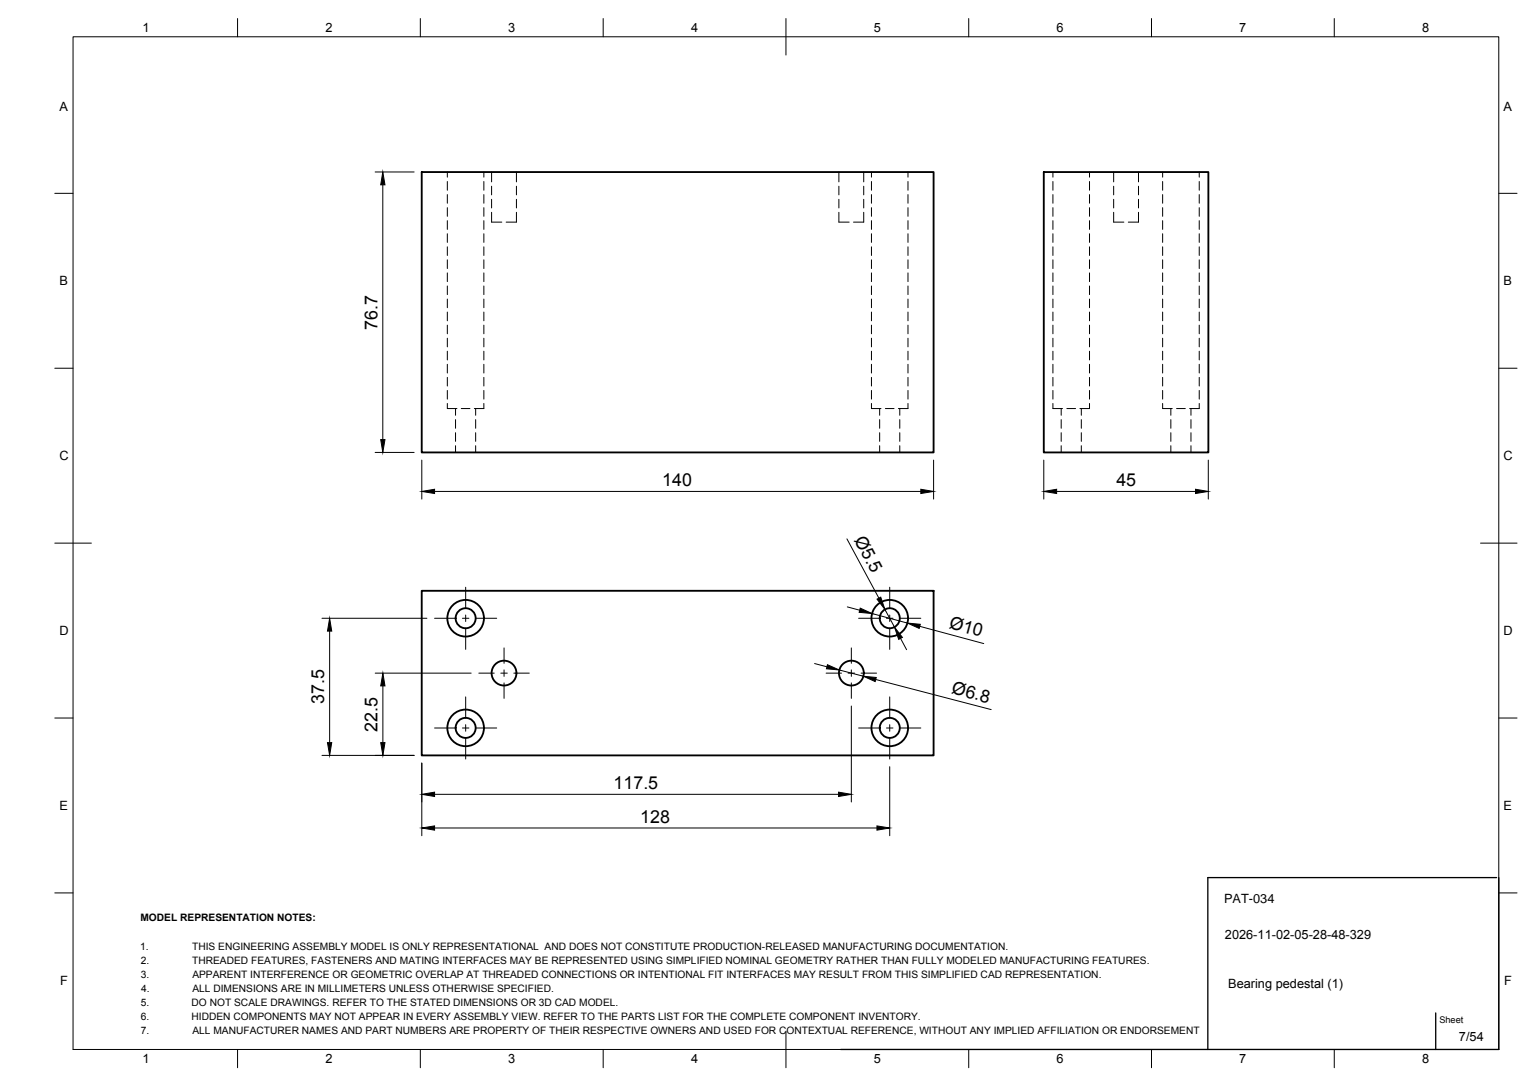
ISO-10303-21;
HEADER;
/* Generated by software containing ST-Developer
 * from STEP Tools, Inc. (www.steptools.com) 
 */

FILE_DESCRIPTION(
/* description */ ('Fatigue rig crank-slider'),
/* implementation_level */ '2;1');

FILE_NAME(
/* name */ 'Bearing pedestal (1).step',
/* time_stamp */ '2026-10-28T03:24:50-07:00',
/* author */ (''),
/* organization */ (''),
/* preprocessor_version */ 'ST-DEVELOPER v20.2',
/* originating_system */ 'Autodesk Translation Framework v15.17.0.0',
/* authorisation */ '');

FILE_SCHEMA (('AUTOMOTIVE_DESIGN { 1 0 10303 214 3 1 1 }'));
ENDSEC;

DATA;
#10=MECHANICAL_DESIGN_GEOMETRIC_PRESENTATION_REPRESENTATION('',(#591),#16911);
#491=SHAPE_REPRESENTATION_RELATIONSHIP('SRR','None',#17130,#541);
#541=ADVANCED_BREP_SHAPE_REPRESENTATION('',(#650),#16859);
#591=STYLED_ITEM('',(#17487),#650);
#650=MANIFOLD_SOLID_BREP('Body1',#8882);
#742=FACE_BOUND('',#1836,.T.);
#743=FACE_BOUND('',#1839,.T.);
#744=FACE_BOUND('',#1842,.T.);
#745=FACE_BOUND('',#1845,.T.);
#746=FACE_BOUND('',#1855,.T.);
#747=FACE_BOUND('',#1856,.T.);
#748=FACE_BOUND('',#1857,.T.);
#749=FACE_BOUND('',#1858,.T.);
#750=FACE_BOUND('',#1859,.T.);
#751=FACE_BOUND('',#1860,.T.);
#752=FACE_BOUND('',#1862,.T.);
#753=FACE_BOUND('',#1863,.T.);
#754=FACE_BOUND('',#1864,.T.);
#755=FACE_BOUND('',#1865,.T.);
#919=PLANE('',#9603);
#920=PLANE('',#9607);
#921=PLANE('',#9611);
#922=PLANE('',#9616);
#923=PLANE('',#9621);
#924=PLANE('',#9626);
#925=PLANE('',#9636);
#926=PLANE('',#9637);
#927=PLANE('',#9638);
#928=PLANE('',#9639);
#929=PLANE('',#9640);
#930=PLANE('',#9641);
#1265=FACE_OUTER_BOUND('',#1830,.T.);
#1266=FACE_OUTER_BOUND('',#1831,.T.);
#1267=FACE_OUTER_BOUND('',#1832,.T.);
#1268=FACE_OUTER_BOUND('',#1833,.T.);
#1269=FACE_OUTER_BOUND('',#1834,.T.);
#1270=FACE_OUTER_BOUND('',#1835,.T.);
#1271=FACE_OUTER_BOUND('',#1837,.T.);
#1272=FACE_OUTER_BOUND('',#1838,.T.);
#1273=FACE_OUTER_BOUND('',#1840,.T.);
#1274=FACE_OUTER_BOUND('',#1841,.T.);
#1275=FACE_OUTER_BOUND('',#1843,.T.);
#1276=FACE_OUTER_BOUND('',#1844,.T.);
#1277=FACE_OUTER_BOUND('',#1846,.T.);
#1278=FACE_OUTER_BOUND('',#1847,.T.);
#1279=FACE_OUTER_BOUND('',#1848,.T.);
#1280=FACE_OUTER_BOUND('',#1849,.T.);
#1281=FACE_OUTER_BOUND('',#1850,.T.);
#1282=FACE_OUTER_BOUND('',#1851,.T.);
#1283=FACE_OUTER_BOUND('',#1852,.T.);
#1284=FACE_OUTER_BOUND('',#1853,.T.);
#1285=FACE_OUTER_BOUND('',#1854,.T.);
#1286=FACE_OUTER_BOUND('',#1861,.T.);
#1830=EDGE_LOOP('',(#6200,#6201,#6202,#6203));
#1831=EDGE_LOOP('',(#6204));
#1832=EDGE_LOOP('',(#6205,#6206,#6207,#6208));
#1833=EDGE_LOOP('',(#6209));
#1834=EDGE_LOOP('',(#6210,#6211,#6212,#6213));
#1835=EDGE_LOOP('',(#6214));
#1836=EDGE_LOOP('',(#6215));
#1837=EDGE_LOOP('',(#6216,#6217,#6218,#6219));
#1838=EDGE_LOOP('',(#6220));
#1839=EDGE_LOOP('',(#6221));
#1840=EDGE_LOOP('',(#6222,#6223,#6224,#6225));
#1841=EDGE_LOOP('',(#6226));
#1842=EDGE_LOOP('',(#6227));
#1843=EDGE_LOOP('',(#6228,#6229,#6230,#6231));
#1844=EDGE_LOOP('',(#6232));
#1845=EDGE_LOOP('',(#6233));
#1846=EDGE_LOOP('',(#6234,#6235,#6236,#6237));
#1847=EDGE_LOOP('',(#6238,#6239,#6240,#6241));
#1848=EDGE_LOOP('',(#6242,#6243,#6244,#6245));
#1849=EDGE_LOOP('',(#6246,#6247,#6248,#6249));
#1850=EDGE_LOOP('',(#6250,#6251,#6252,#6253));
#1851=EDGE_LOOP('',(#6254,#6255,#6256,#6257));
#1852=EDGE_LOOP('',(#6258,#6259,#6260,#6261));
#1853=EDGE_LOOP('',(#6262,#6263,#6264,#6265));
#1854=EDGE_LOOP('',(#6266,#6267,#6268,#6269));
#1855=EDGE_LOOP('',(#6270));
#1856=EDGE_LOOP('',(#6271));
#1857=EDGE_LOOP('',(#6272));
#1858=EDGE_LOOP('',(#6273));
#1859=EDGE_LOOP('',(#6274));
#1860=EDGE_LOOP('',(#6275));
#1861=EDGE_LOOP('',(#6276,#6277,#6278,#6279));
#1862=EDGE_LOOP('',(#6280));
#1863=EDGE_LOOP('',(#6281));
#1864=EDGE_LOOP('',(#6282));
#1865=EDGE_LOOP('',(#6283));
#2510=LINE('',#13587,#3156);
#2511=LINE('',#13594,#3157);
#2512=LINE('',#13601,#3158);
#2513=LINE('',#13610,#3159);
#2514=LINE('',#13619,#3160);
#2515=LINE('',#13628,#3161);
#2516=LINE('',#13636,#3162);
#2517=LINE('',#13640,#3163);
#2518=LINE('',#13644,#3164);
#2519=LINE('',#13648,#3165);
#2520=LINE('',#13652,#3166);
#2521=LINE('',#13654,#3167);
#2522=LINE('',#13656,#3168);
#2523=LINE('',#13657,#3169);
#2524=LINE('',#13660,#3170);
#2525=LINE('',#13662,#3171);
#2526=LINE('',#13663,#3172);
#2527=LINE('',#13666,#3173);
#2528=LINE('',#13668,#3174);
#2529=LINE('',#13669,#3175);
#2530=LINE('',#13671,#3176);
#2531=LINE('',#13672,#3177);
#3156=VECTOR('',#10834,0.34);
#3157=VECTOR('',#10843,0.34);
#3158=VECTOR('',#10852,0.5);
#3159=VECTOR('',#10863,0.5);
#3160=VECTOR('',#10874,0.5);
#3161=VECTOR('',#10885,0.5);
#3162=VECTOR('',#10896,0.275);
#3163=VECTOR('',#10901,0.275);
#3164=VECTOR('',#10906,0.275);
#3165=VECTOR('',#10911,0.275);
#3166=VECTOR('',#10914,1.);
#3167=VECTOR('',#10915,1.);
#3168=VECTOR('',#10916,1.);
#3169=VECTOR('',#10917,1.);
#3170=VECTOR('',#10920,1.);
#3171=VECTOR('',#10921,1.);
#3172=VECTOR('',#10922,1.);
#3173=VECTOR('',#10925,1.);
#3174=VECTOR('',#10926,1.);
#3175=VECTOR('',#10927,1.);
#3176=VECTOR('',#10930,1.);
#3177=VECTOR('',#10931,1.);
#3804=CIRCLE('',#9601,0.34);
#3805=CIRCLE('',#9602,0.34);
#3806=CIRCLE('',#9605,0.34);
#3807=CIRCLE('',#9606,0.34);
#3808=CIRCLE('',#9609,0.5);
#3809=CIRCLE('',#9610,0.5);
#3810=CIRCLE('',#9612,0.275);
#3811=CIRCLE('',#9614,0.5);
#3812=CIRCLE('',#9615,0.5);
#3813=CIRCLE('',#9617,0.275);
#3814=CIRCLE('',#9619,0.5);
#3815=CIRCLE('',#9620,0.5);
#3816=CIRCLE('',#9622,0.275);
#3817=CIRCLE('',#9624,0.5);
#3818=CIRCLE('',#9625,0.5);
#3819=CIRCLE('',#9627,0.275);
#3820=CIRCLE('',#9629,0.275);
#3821=CIRCLE('',#9631,0.275);
#3822=CIRCLE('',#9633,0.275);
#3823=CIRCLE('',#9635,0.275);
#4220=VERTEX_POINT('',#13584);
#4221=VERTEX_POINT('',#13586);
#4222=VERTEX_POINT('',#13591);
#4223=VERTEX_POINT('',#13593);
#4224=VERTEX_POINT('',#13598);
#4225=VERTEX_POINT('',#13600);
#4226=VERTEX_POINT('',#13604);
#4227=VERTEX_POINT('',#13607);
#4228=VERTEX_POINT('',#13609);
#4229=VERTEX_POINT('',#13613);
#4230=VERTEX_POINT('',#13616);
#4231=VERTEX_POINT('',#13618);
#4232=VERTEX_POINT('',#13622);
#4233=VERTEX_POINT('',#13625);
#4234=VERTEX_POINT('',#13627);
#4235=VERTEX_POINT('',#13631);
#4236=VERTEX_POINT('',#13634);
#4237=VERTEX_POINT('',#13638);
#4238=VERTEX_POINT('',#13642);
#4239=VERTEX_POINT('',#13646);
#4240=VERTEX_POINT('',#13650);
#4241=VERTEX_POINT('',#13651);
#4242=VERTEX_POINT('',#13653);
#4243=VERTEX_POINT('',#13655);
#4244=VERTEX_POINT('',#13659);
#4245=VERTEX_POINT('',#13661);
#4246=VERTEX_POINT('',#13665);
#4247=VERTEX_POINT('',#13667);
#4998=EDGE_CURVE('',#4220,#4220,#3804,.T.);
#4999=EDGE_CURVE('',#4220,#4221,#2510,.T.);
#5000=EDGE_CURVE('',#4221,#4221,#3805,.T.);
#5001=EDGE_CURVE('',#4222,#4222,#3806,.T.);
#5002=EDGE_CURVE('',#4222,#4223,#2511,.T.);
#5003=EDGE_CURVE('',#4223,#4223,#3807,.T.);
#5004=EDGE_CURVE('',#4224,#4224,#3808,.T.);
#5005=EDGE_CURVE('',#4224,#4225,#2512,.T.);
#5006=EDGE_CURVE('',#4225,#4225,#3809,.T.);
#5007=EDGE_CURVE('',#4226,#4226,#3810,.T.);
#5008=EDGE_CURVE('',#4227,#4227,#3811,.T.);
#5009=EDGE_CURVE('',#4227,#4228,#2513,.T.);
#5010=EDGE_CURVE('',#4228,#4228,#3812,.T.);
#5011=EDGE_CURVE('',#4229,#4229,#3813,.T.);
#5012=EDGE_CURVE('',#4230,#4230,#3814,.T.);
#5013=EDGE_CURVE('',#4230,#4231,#2514,.T.);
#5014=EDGE_CURVE('',#4231,#4231,#3815,.T.);
#5015=EDGE_CURVE('',#4232,#4232,#3816,.T.);
#5016=EDGE_CURVE('',#4233,#4233,#3817,.T.);
#5017=EDGE_CURVE('',#4233,#4234,#2515,.T.);
#5018=EDGE_CURVE('',#4234,#4234,#3818,.T.);
#5019=EDGE_CURVE('',#4235,#4235,#3819,.T.);
#5020=EDGE_CURVE('',#4236,#4236,#3820,.T.);
#5021=EDGE_CURVE('',#4236,#4226,#2516,.T.);
#5022=EDGE_CURVE('',#4237,#4237,#3821,.T.);
#5023=EDGE_CURVE('',#4237,#4229,#2517,.T.);
#5024=EDGE_CURVE('',#4238,#4238,#3822,.T.);
#5025=EDGE_CURVE('',#4238,#4232,#2518,.T.);
#5026=EDGE_CURVE('',#4239,#4239,#3823,.T.);
#5027=EDGE_CURVE('',#4239,#4235,#2519,.T.);
#5028=EDGE_CURVE('',#4240,#4241,#2520,.T.);
#5029=EDGE_CURVE('',#4241,#4242,#2521,.T.);
#5030=EDGE_CURVE('',#4243,#4242,#2522,.T.);
#5031=EDGE_CURVE('',#4240,#4243,#2523,.T.);
#5032=EDGE_CURVE('',#4244,#4240,#2524,.T.);
#5033=EDGE_CURVE('',#4245,#4243,#2525,.T.);
#5034=EDGE_CURVE('',#4244,#4245,#2526,.T.);
#5035=EDGE_CURVE('',#4246,#4244,#2527,.T.);
#5036=EDGE_CURVE('',#4247,#4245,#2528,.T.);
#5037=EDGE_CURVE('',#4246,#4247,#2529,.T.);
#5038=EDGE_CURVE('',#4241,#4246,#2530,.T.);
#5039=EDGE_CURVE('',#4242,#4247,#2531,.T.);
#6200=ORIENTED_EDGE('',*,*,#4998,.F.);
#6201=ORIENTED_EDGE('',*,*,#4999,.T.);
#6202=ORIENTED_EDGE('',*,*,#5000,.F.);
#6203=ORIENTED_EDGE('',*,*,#4999,.F.);
#6204=ORIENTED_EDGE('',*,*,#4998,.T.);
#6205=ORIENTED_EDGE('',*,*,#5001,.F.);
#6206=ORIENTED_EDGE('',*,*,#5002,.T.);
#6207=ORIENTED_EDGE('',*,*,#5003,.F.);
#6208=ORIENTED_EDGE('',*,*,#5002,.F.);
#6209=ORIENTED_EDGE('',*,*,#5001,.T.);
#6210=ORIENTED_EDGE('',*,*,#5004,.F.);
#6211=ORIENTED_EDGE('',*,*,#5005,.T.);
#6212=ORIENTED_EDGE('',*,*,#5006,.F.);
#6213=ORIENTED_EDGE('',*,*,#5005,.F.);
#6214=ORIENTED_EDGE('',*,*,#5004,.T.);
#6215=ORIENTED_EDGE('',*,*,#5007,.F.);
#6216=ORIENTED_EDGE('',*,*,#5008,.F.);
#6217=ORIENTED_EDGE('',*,*,#5009,.T.);
#6218=ORIENTED_EDGE('',*,*,#5010,.F.);
#6219=ORIENTED_EDGE('',*,*,#5009,.F.);
#6220=ORIENTED_EDGE('',*,*,#5008,.T.);
#6221=ORIENTED_EDGE('',*,*,#5011,.F.);
#6222=ORIENTED_EDGE('',*,*,#5012,.F.);
#6223=ORIENTED_EDGE('',*,*,#5013,.T.);
#6224=ORIENTED_EDGE('',*,*,#5014,.F.);
#6225=ORIENTED_EDGE('',*,*,#5013,.F.);
#6226=ORIENTED_EDGE('',*,*,#5012,.T.);
#6227=ORIENTED_EDGE('',*,*,#5015,.F.);
#6228=ORIENTED_EDGE('',*,*,#5016,.F.);
#6229=ORIENTED_EDGE('',*,*,#5017,.T.);
#6230=ORIENTED_EDGE('',*,*,#5018,.F.);
#6231=ORIENTED_EDGE('',*,*,#5017,.F.);
#6232=ORIENTED_EDGE('',*,*,#5016,.T.);
#6233=ORIENTED_EDGE('',*,*,#5019,.F.);
#6234=ORIENTED_EDGE('',*,*,#5020,.F.);
#6235=ORIENTED_EDGE('',*,*,#5021,.T.);
#6236=ORIENTED_EDGE('',*,*,#5007,.T.);
#6237=ORIENTED_EDGE('',*,*,#5021,.F.);
#6238=ORIENTED_EDGE('',*,*,#5022,.F.);
#6239=ORIENTED_EDGE('',*,*,#5023,.T.);
#6240=ORIENTED_EDGE('',*,*,#5011,.T.);
#6241=ORIENTED_EDGE('',*,*,#5023,.F.);
#6242=ORIENTED_EDGE('',*,*,#5024,.F.);
#6243=ORIENTED_EDGE('',*,*,#5025,.T.);
#6244=ORIENTED_EDGE('',*,*,#5015,.T.);
#6245=ORIENTED_EDGE('',*,*,#5025,.F.);
#6246=ORIENTED_EDGE('',*,*,#5026,.F.);
#6247=ORIENTED_EDGE('',*,*,#5027,.T.);
#6248=ORIENTED_EDGE('',*,*,#5019,.T.);
#6249=ORIENTED_EDGE('',*,*,#5027,.F.);
#6250=ORIENTED_EDGE('',*,*,#5028,.T.);
#6251=ORIENTED_EDGE('',*,*,#5029,.T.);
#6252=ORIENTED_EDGE('',*,*,#5030,.F.);
#6253=ORIENTED_EDGE('',*,*,#5031,.F.);
#6254=ORIENTED_EDGE('',*,*,#5032,.T.);
#6255=ORIENTED_EDGE('',*,*,#5031,.T.);
#6256=ORIENTED_EDGE('',*,*,#5033,.F.);
#6257=ORIENTED_EDGE('',*,*,#5034,.F.);
#6258=ORIENTED_EDGE('',*,*,#5035,.T.);
#6259=ORIENTED_EDGE('',*,*,#5034,.T.);
#6260=ORIENTED_EDGE('',*,*,#5036,.F.);
#6261=ORIENTED_EDGE('',*,*,#5037,.F.);
#6262=ORIENTED_EDGE('',*,*,#5038,.T.);
#6263=ORIENTED_EDGE('',*,*,#5037,.T.);
#6264=ORIENTED_EDGE('',*,*,#5039,.F.);
#6265=ORIENTED_EDGE('',*,*,#5029,.F.);
#6266=ORIENTED_EDGE('',*,*,#5039,.T.);
#6267=ORIENTED_EDGE('',*,*,#5036,.T.);
#6268=ORIENTED_EDGE('',*,*,#5033,.T.);
#6269=ORIENTED_EDGE('',*,*,#5030,.T.);
#6270=ORIENTED_EDGE('',*,*,#5000,.T.);
#6271=ORIENTED_EDGE('',*,*,#5003,.T.);
#6272=ORIENTED_EDGE('',*,*,#5018,.T.);
#6273=ORIENTED_EDGE('',*,*,#5014,.T.);
#6274=ORIENTED_EDGE('',*,*,#5010,.T.);
#6275=ORIENTED_EDGE('',*,*,#5006,.T.);
#6276=ORIENTED_EDGE('',*,*,#5038,.F.);
#6277=ORIENTED_EDGE('',*,*,#5028,.F.);
#6278=ORIENTED_EDGE('',*,*,#5032,.F.);
#6279=ORIENTED_EDGE('',*,*,#5035,.F.);
#6280=ORIENTED_EDGE('',*,*,#5020,.T.);
#6281=ORIENTED_EDGE('',*,*,#5022,.T.);
#6282=ORIENTED_EDGE('',*,*,#5024,.T.);
#6283=ORIENTED_EDGE('',*,*,#5026,.T.);
#8222=CYLINDRICAL_SURFACE('',#9600,0.34);
#8223=CYLINDRICAL_SURFACE('',#9604,0.34);
#8224=CYLINDRICAL_SURFACE('',#9608,0.5);
#8225=CYLINDRICAL_SURFACE('',#9613,0.5);
#8226=CYLINDRICAL_SURFACE('',#9618,0.5);
#8227=CYLINDRICAL_SURFACE('',#9623,0.5);
#8228=CYLINDRICAL_SURFACE('',#9628,0.275);
#8229=CYLINDRICAL_SURFACE('',#9630,0.275);
#8230=CYLINDRICAL_SURFACE('',#9632,0.275);
#8231=CYLINDRICAL_SURFACE('',#9634,0.275);
#8403=ADVANCED_FACE('',(#1265),#8222,.F.);
#8404=ADVANCED_FACE('',(#1266),#919,.T.);
#8405=ADVANCED_FACE('',(#1267),#8223,.F.);
#8406=ADVANCED_FACE('',(#1268),#920,.T.);
#8407=ADVANCED_FACE('',(#1269),#8224,.F.);
#8408=ADVANCED_FACE('',(#1270,#742),#921,.T.);
#8409=ADVANCED_FACE('',(#1271),#8225,.F.);
#8410=ADVANCED_FACE('',(#1272,#743),#922,.T.);
#8411=ADVANCED_FACE('',(#1273),#8226,.F.);
#8412=ADVANCED_FACE('',(#1274,#744),#923,.T.);
#8413=ADVANCED_FACE('',(#1275),#8227,.F.);
#8414=ADVANCED_FACE('',(#1276,#745),#924,.T.);
#8415=ADVANCED_FACE('',(#1277),#8228,.F.);
#8416=ADVANCED_FACE('',(#1278),#8229,.F.);
#8417=ADVANCED_FACE('',(#1279),#8230,.F.);
#8418=ADVANCED_FACE('',(#1280),#8231,.F.);
#8419=ADVANCED_FACE('',(#1281),#925,.T.);
#8420=ADVANCED_FACE('',(#1282),#926,.T.);
#8421=ADVANCED_FACE('',(#1283),#927,.T.);
#8422=ADVANCED_FACE('',(#1284),#928,.T.);
#8423=ADVANCED_FACE('',(#1285,#746,#747,#748,#749,#750,#751),#929,.T.);
#8424=ADVANCED_FACE('',(#1286,#752,#753,#754,#755),#930,.F.);
#8882=CLOSED_SHELL('',(#8403,#8404,#8405,#8406,#8407,#8408,#8409,#8410,
#8411,#8412,#8413,#8414,#8415,#8416,#8417,#8418,#8419,#8420,#8421,#8422,
#8423,#8424));
#9599=AXIS2_PLACEMENT_3D('',#13582,#10828,#10829);
#9600=AXIS2_PLACEMENT_3D('',#13583,#10830,#10831);
#9601=AXIS2_PLACEMENT_3D('',#13585,#10832,#10833);
#9602=AXIS2_PLACEMENT_3D('',#13588,#10835,#10836);
#9603=AXIS2_PLACEMENT_3D('',#13589,#10837,#10838);
#9604=AXIS2_PLACEMENT_3D('',#13590,#10839,#10840);
#9605=AXIS2_PLACEMENT_3D('',#13592,#10841,#10842);
#9606=AXIS2_PLACEMENT_3D('',#13595,#10844,#10845);
#9607=AXIS2_PLACEMENT_3D('',#13596,#10846,#10847);
#9608=AXIS2_PLACEMENT_3D('',#13597,#10848,#10849);
#9609=AXIS2_PLACEMENT_3D('',#13599,#10850,#10851);
#9610=AXIS2_PLACEMENT_3D('',#13602,#10853,#10854);
#9611=AXIS2_PLACEMENT_3D('',#13603,#10855,#10856);
#9612=AXIS2_PLACEMENT_3D('',#13605,#10857,#10858);
#9613=AXIS2_PLACEMENT_3D('',#13606,#10859,#10860);
#9614=AXIS2_PLACEMENT_3D('',#13608,#10861,#10862);
#9615=AXIS2_PLACEMENT_3D('',#13611,#10864,#10865);
#9616=AXIS2_PLACEMENT_3D('',#13612,#10866,#10867);
#9617=AXIS2_PLACEMENT_3D('',#13614,#10868,#10869);
#9618=AXIS2_PLACEMENT_3D('',#13615,#10870,#10871);
#9619=AXIS2_PLACEMENT_3D('',#13617,#10872,#10873);
#9620=AXIS2_PLACEMENT_3D('',#13620,#10875,#10876);
#9621=AXIS2_PLACEMENT_3D('',#13621,#10877,#10878);
#9622=AXIS2_PLACEMENT_3D('',#13623,#10879,#10880);
#9623=AXIS2_PLACEMENT_3D('',#13624,#10881,#10882);
#9624=AXIS2_PLACEMENT_3D('',#13626,#10883,#10884);
#9625=AXIS2_PLACEMENT_3D('',#13629,#10886,#10887);
#9626=AXIS2_PLACEMENT_3D('',#13630,#10888,#10889);
#9627=AXIS2_PLACEMENT_3D('',#13632,#10890,#10891);
#9628=AXIS2_PLACEMENT_3D('',#13633,#10892,#10893);
#9629=AXIS2_PLACEMENT_3D('',#13635,#10894,#10895);
#9630=AXIS2_PLACEMENT_3D('',#13637,#10897,#10898);
#9631=AXIS2_PLACEMENT_3D('',#13639,#10899,#10900);
#9632=AXIS2_PLACEMENT_3D('',#13641,#10902,#10903);
#9633=AXIS2_PLACEMENT_3D('',#13643,#10904,#10905);
#9634=AXIS2_PLACEMENT_3D('',#13645,#10907,#10908);
#9635=AXIS2_PLACEMENT_3D('',#13647,#10909,#10910);
#9636=AXIS2_PLACEMENT_3D('',#13649,#10912,#10913);
#9637=AXIS2_PLACEMENT_3D('',#13658,#10918,#10919);
#9638=AXIS2_PLACEMENT_3D('',#13664,#10923,#10924);
#9639=AXIS2_PLACEMENT_3D('',#13670,#10928,#10929);
#9640=AXIS2_PLACEMENT_3D('',#13673,#10932,#10933);
#9641=AXIS2_PLACEMENT_3D('',#13674,#10934,#10935);
#10828=DIRECTION('axis',(0.,0.,1.));
#10829=DIRECTION('refdir',(1.,0.,0.));
#10830=DIRECTION('center_axis',(0.,0.,1.));
#10831=DIRECTION('ref_axis',(1.,0.,0.));
#10832=DIRECTION('center_axis',(0.,0.,1.));
#10833=DIRECTION('ref_axis',(1.,0.,0.));
#10834=DIRECTION('',(0.,0.,1.));
#10835=DIRECTION('center_axis',(0.,0.,-1.));
#10836=DIRECTION('ref_axis',(1.,0.,0.));
#10837=DIRECTION('center_axis',(0.,0.,1.));
#10838=DIRECTION('ref_axis',(1.,0.,0.));
#10839=DIRECTION('center_axis',(0.,0.,1.));
#10840=DIRECTION('ref_axis',(1.,0.,0.));
#10841=DIRECTION('center_axis',(0.,0.,1.));
#10842=DIRECTION('ref_axis',(1.,0.,0.));
#10843=DIRECTION('',(0.,0.,1.));
#10844=DIRECTION('center_axis',(0.,0.,-1.));
#10845=DIRECTION('ref_axis',(1.,0.,0.));
#10846=DIRECTION('center_axis',(0.,0.,1.));
#10847=DIRECTION('ref_axis',(1.,0.,0.));
#10848=DIRECTION('center_axis',(0.,0.,1.));
#10849=DIRECTION('ref_axis',(1.,0.,0.));
#10850=DIRECTION('center_axis',(0.,0.,1.));
#10851=DIRECTION('ref_axis',(1.,0.,0.));
#10852=DIRECTION('',(0.,0.,1.));
#10853=DIRECTION('center_axis',(0.,0.,-1.));
#10854=DIRECTION('ref_axis',(1.,0.,0.));
#10855=DIRECTION('center_axis',(0.,0.,1.));
#10856=DIRECTION('ref_axis',(1.,0.,0.));
#10857=DIRECTION('center_axis',(0.,0.,1.));
#10858=DIRECTION('ref_axis',(1.,0.,0.));
#10859=DIRECTION('center_axis',(0.,0.,1.));
#10860=DIRECTION('ref_axis',(1.,0.,0.));
#10861=DIRECTION('center_axis',(0.,0.,1.));
#10862=DIRECTION('ref_axis',(1.,0.,0.));
#10863=DIRECTION('',(0.,0.,1.));
#10864=DIRECTION('center_axis',(0.,0.,-1.));
#10865=DIRECTION('ref_axis',(1.,0.,0.));
#10866=DIRECTION('center_axis',(0.,0.,1.));
#10867=DIRECTION('ref_axis',(1.,0.,0.));
#10868=DIRECTION('center_axis',(0.,0.,1.));
#10869=DIRECTION('ref_axis',(1.,0.,0.));
#10870=DIRECTION('center_axis',(0.,0.,1.));
#10871=DIRECTION('ref_axis',(1.,0.,0.));
#10872=DIRECTION('center_axis',(0.,0.,1.));
#10873=DIRECTION('ref_axis',(1.,0.,0.));
#10874=DIRECTION('',(0.,0.,1.));
#10875=DIRECTION('center_axis',(0.,0.,-1.));
#10876=DIRECTION('ref_axis',(1.,0.,0.));
#10877=DIRECTION('center_axis',(0.,0.,1.));
#10878=DIRECTION('ref_axis',(1.,0.,0.));
#10879=DIRECTION('center_axis',(0.,0.,1.));
#10880=DIRECTION('ref_axis',(1.,0.,0.));
#10881=DIRECTION('center_axis',(0.,0.,1.));
#10882=DIRECTION('ref_axis',(1.,0.,0.));
#10883=DIRECTION('center_axis',(0.,0.,1.));
#10884=DIRECTION('ref_axis',(1.,0.,0.));
#10885=DIRECTION('',(0.,0.,1.));
#10886=DIRECTION('center_axis',(0.,0.,-1.));
#10887=DIRECTION('ref_axis',(1.,0.,0.));
#10888=DIRECTION('center_axis',(0.,0.,1.));
#10889=DIRECTION('ref_axis',(1.,0.,0.));
#10890=DIRECTION('center_axis',(0.,0.,1.));
#10891=DIRECTION('ref_axis',(1.,0.,0.));
#10892=DIRECTION('center_axis',(0.,0.,1.));
#10893=DIRECTION('ref_axis',(1.,0.,0.));
#10894=DIRECTION('center_axis',(0.,0.,1.));
#10895=DIRECTION('ref_axis',(1.,0.,0.));
#10896=DIRECTION('',(0.,0.,1.));
#10897=DIRECTION('center_axis',(0.,0.,1.));
#10898=DIRECTION('ref_axis',(1.,0.,0.));
#10899=DIRECTION('center_axis',(0.,0.,1.));
#10900=DIRECTION('ref_axis',(1.,0.,0.));
#10901=DIRECTION('',(0.,0.,1.));
#10902=DIRECTION('center_axis',(0.,0.,1.));
#10903=DIRECTION('ref_axis',(1.,0.,0.));
#10904=DIRECTION('center_axis',(0.,0.,1.));
#10905=DIRECTION('ref_axis',(1.,0.,0.));
#10906=DIRECTION('',(0.,0.,1.));
#10907=DIRECTION('center_axis',(0.,0.,1.));
#10908=DIRECTION('ref_axis',(1.,0.,0.));
#10909=DIRECTION('center_axis',(0.,0.,1.));
#10910=DIRECTION('ref_axis',(1.,0.,0.));
#10911=DIRECTION('',(0.,0.,1.));
#10912=DIRECTION('center_axis',(0.,1.,0.));
#10913=DIRECTION('ref_axis',(-1.,0.,0.));
#10914=DIRECTION('',(-1.,0.,0.));
#10915=DIRECTION('',(0.,0.,1.));
#10916=DIRECTION('',(-1.,0.,0.));
#10917=DIRECTION('',(0.,0.,1.));
#10918=DIRECTION('center_axis',(1.,0.,0.));
#10919=DIRECTION('ref_axis',(0.,1.,0.));
#10920=DIRECTION('',(0.,1.,0.));
#10921=DIRECTION('',(0.,1.,0.));
#10922=DIRECTION('',(0.,0.,1.));
#10923=DIRECTION('center_axis',(0.,-1.,0.));
#10924=DIRECTION('ref_axis',(1.,0.,0.));
#10925=DIRECTION('',(1.,0.,0.));
#10926=DIRECTION('',(1.,0.,0.));
#10927=DIRECTION('',(0.,0.,1.));
#10928=DIRECTION('center_axis',(-1.,0.,0.));
#10929=DIRECTION('ref_axis',(0.,-1.,0.));
#10930=DIRECTION('',(0.,-1.,0.));
#10931=DIRECTION('',(0.,-1.,0.));
#10932=DIRECTION('center_axis',(0.,0.,1.));
#10933=DIRECTION('ref_axis',(1.,0.,0.));
#10934=DIRECTION('center_axis',(0.,0.,1.));
#10935=DIRECTION('ref_axis',(1.,0.,0.));
#13582=CARTESIAN_POINT('',(0.,0.,0.));
#13583=CARTESIAN_POINT('Origin',(-4.75,-7.,7.3));
#13584=CARTESIAN_POINT('',(-5.09,-7.,7.3));
#13585=CARTESIAN_POINT('Origin',(-4.75,-7.,7.3));
#13586=CARTESIAN_POINT('',(-5.09,-7.,8.67));
#13587=CARTESIAN_POINT('',(-5.09,-7.,7.3));
#13588=CARTESIAN_POINT('Origin',(-4.75,-7.,8.67));
#13589=CARTESIAN_POINT('Origin',(-4.75,-7.,7.3));
#13590=CARTESIAN_POINT('Origin',(4.75,-7.,7.3));
#13591=CARTESIAN_POINT('',(4.41,-7.,7.3));
#13592=CARTESIAN_POINT('Origin',(4.75,-7.,7.3));
#13593=CARTESIAN_POINT('',(4.41,-7.,8.67));
#13594=CARTESIAN_POINT('',(4.41,-7.,7.3));
#13595=CARTESIAN_POINT('Origin',(4.75,-7.,8.67));
#13596=CARTESIAN_POINT('Origin',(4.75,-7.,7.3));
#13597=CARTESIAN_POINT('Origin',(5.8,-8.5,2.2));
#13598=CARTESIAN_POINT('',(5.3,-8.5,2.2));
#13599=CARTESIAN_POINT('Origin',(5.8,-8.5,2.2));
#13600=CARTESIAN_POINT('',(5.3,-8.5,8.67));
#13601=CARTESIAN_POINT('',(5.3,-8.5,2.2));
#13602=CARTESIAN_POINT('Origin',(5.8,-8.5,8.67));
#13603=CARTESIAN_POINT('Origin',(5.8,-8.5,2.2));
#13604=CARTESIAN_POINT('',(5.525,-8.5,2.2));
#13605=CARTESIAN_POINT('Origin',(5.8,-8.5,2.2));
#13606=CARTESIAN_POINT('Origin',(-5.8,-5.5,2.2));
#13607=CARTESIAN_POINT('',(-6.3,-5.5,2.2));
#13608=CARTESIAN_POINT('Origin',(-5.8,-5.5,2.2));
#13609=CARTESIAN_POINT('',(-6.3,-5.5,8.67));
#13610=CARTESIAN_POINT('',(-6.3,-5.5,2.2));
#13611=CARTESIAN_POINT('Origin',(-5.8,-5.5,8.67));
#13612=CARTESIAN_POINT('Origin',(-5.8,-5.5,2.2));
#13613=CARTESIAN_POINT('',(-6.075,-5.5,2.2));
#13614=CARTESIAN_POINT('Origin',(-5.8,-5.5,2.2));
#13615=CARTESIAN_POINT('Origin',(-5.8,-8.5,2.2));
#13616=CARTESIAN_POINT('',(-6.3,-8.5,2.2));
#13617=CARTESIAN_POINT('Origin',(-5.8,-8.5,2.2));
#13618=CARTESIAN_POINT('',(-6.3,-8.5,8.67));
#13619=CARTESIAN_POINT('',(-6.3,-8.5,2.2));
#13620=CARTESIAN_POINT('Origin',(-5.8,-8.5,8.67));
#13621=CARTESIAN_POINT('Origin',(-5.8,-8.5,2.2));
#13622=CARTESIAN_POINT('',(-6.075,-8.5,2.2));
#13623=CARTESIAN_POINT('Origin',(-5.8,-8.5,2.2));
#13624=CARTESIAN_POINT('Origin',(5.8,-5.5,2.2));
#13625=CARTESIAN_POINT('',(5.3,-5.5,2.2));
#13626=CARTESIAN_POINT('Origin',(5.8,-5.5,2.2));
#13627=CARTESIAN_POINT('',(5.3,-5.5,8.67));
#13628=CARTESIAN_POINT('',(5.3,-5.5,2.2));
#13629=CARTESIAN_POINT('Origin',(5.8,-5.5,8.67));
#13630=CARTESIAN_POINT('Origin',(5.8,-5.5,2.2));
#13631=CARTESIAN_POINT('',(5.525,-5.5,2.2));
#13632=CARTESIAN_POINT('Origin',(5.8,-5.5,2.2));
#13633=CARTESIAN_POINT('Origin',(5.8,-8.5,0.9));
#13634=CARTESIAN_POINT('',(5.525,-8.5,1.));
#13635=CARTESIAN_POINT('Origin',(5.8,-8.5,1.));
#13636=CARTESIAN_POINT('',(5.525,-8.5,0.9));
#13637=CARTESIAN_POINT('Origin',(-5.8,-5.5,0.9));
#13638=CARTESIAN_POINT('',(-6.075,-5.5,1.));
#13639=CARTESIAN_POINT('Origin',(-5.8,-5.5,1.));
#13640=CARTESIAN_POINT('',(-6.075,-5.5,0.9));
#13641=CARTESIAN_POINT('Origin',(-5.8,-8.5,0.9));
#13642=CARTESIAN_POINT('',(-6.075,-8.5,1.));
#13643=CARTESIAN_POINT('Origin',(-5.8,-8.5,1.));
#13644=CARTESIAN_POINT('',(-6.075,-8.5,0.9));
#13645=CARTESIAN_POINT('Origin',(5.8,-5.5,0.9));
#13646=CARTESIAN_POINT('',(5.525,-5.5,1.));
#13647=CARTESIAN_POINT('Origin',(5.8,-5.5,1.));
#13648=CARTESIAN_POINT('',(5.525,-5.5,0.9));
#13649=CARTESIAN_POINT('Origin',(7.,-4.75,1.));
#13650=CARTESIAN_POINT('',(7.,-4.75,1.));
#13651=CARTESIAN_POINT('',(-7.,-4.75,1.));
#13652=CARTESIAN_POINT('',(7.,-4.75,1.));
#13653=CARTESIAN_POINT('',(-7.,-4.75,8.67));
#13654=CARTESIAN_POINT('',(-7.,-4.75,1.));
#13655=CARTESIAN_POINT('',(7.,-4.75,8.67));
#13656=CARTESIAN_POINT('',(7.,-4.75,8.67));
#13657=CARTESIAN_POINT('',(7.,-4.75,1.));
#13658=CARTESIAN_POINT('Origin',(7.,-9.25,1.));
#13659=CARTESIAN_POINT('',(7.,-9.25,1.));
#13660=CARTESIAN_POINT('',(7.,-9.25,1.));
#13661=CARTESIAN_POINT('',(7.,-9.25,8.67));
#13662=CARTESIAN_POINT('',(7.,-9.25,8.67));
#13663=CARTESIAN_POINT('',(7.,-9.25,1.));
#13664=CARTESIAN_POINT('Origin',(-7.,-9.25,1.));
#13665=CARTESIAN_POINT('',(-7.,-9.25,1.));
#13666=CARTESIAN_POINT('',(-7.,-9.25,1.));
#13667=CARTESIAN_POINT('',(-7.,-9.25,8.67));
#13668=CARTESIAN_POINT('',(-7.,-9.25,8.67));
#13669=CARTESIAN_POINT('',(-7.,-9.25,1.));
#13670=CARTESIAN_POINT('Origin',(-7.,-4.75,1.));
#13671=CARTESIAN_POINT('',(-7.,-4.75,1.));
#13672=CARTESIAN_POINT('',(-7.,-4.75,8.67));
#13673=CARTESIAN_POINT('Origin',(0.,-7.,8.67));
#13674=CARTESIAN_POINT('Origin',(0.,-7.,1.));
#16800=UNCERTAINTY_MEASURE_WITH_UNIT(LENGTH_MEASURE(0.001),#16912,
'DISTANCE_ACCURACY_VALUE',
'Maximum model space distance between geometric entities at asserted c
onnectivities');
#16852=UNCERTAINTY_MEASURE_WITH_UNIT(LENGTH_MEASURE(0.001),#16912,
'DISTANCE_ACCURACY_VALUE',
'Maximum model space distance between geometric entities at asserted c
onnectivities');
#16859=(
GEOMETRIC_REPRESENTATION_CONTEXT(3)
GLOBAL_UNCERTAINTY_ASSIGNED_CONTEXT((#16800))
GLOBAL_UNIT_ASSIGNED_CONTEXT((#16912,#16914,#16915))
REPRESENTATION_CONTEXT('','3D')
);
#16911=(
GEOMETRIC_REPRESENTATION_CONTEXT(3)
GLOBAL_UNCERTAINTY_ASSIGNED_CONTEXT((#16852))
GLOBAL_UNIT_ASSIGNED_CONTEXT((#16912,#16914,#16915))
REPRESENTATION_CONTEXT('','3D')
);
#16912=(
LENGTH_UNIT()
NAMED_UNIT(*)
SI_UNIT(.CENTI.,.METRE.)
);
#16914=(
NAMED_UNIT(*)
PLANE_ANGLE_UNIT()
SI_UNIT($,.RADIAN.)
);
#16915=(
NAMED_UNIT(*)
SI_UNIT($,.STERADIAN.)
SOLID_ANGLE_UNIT()
);
#16922=SHAPE_DEFINITION_REPRESENTATION(#16980,#17130);
#16980=PRODUCT_DEFINITION_SHAPE('',$,#17189);
#17130=SHAPE_REPRESENTATION('',(#9599),#16859);
#17182=PRODUCT_DEFINITION_CONTEXT('part definition',#17358,'design');
#17189=PRODUCT_DEFINITION('Bearing pedestal (1)','Bearing pedestal (1)',#17247,
#17182);
#17247=PRODUCT_DEFINITION_FORMATION('',$,#17366);
#17358=APPLICATION_CONTEXT(
'Core Data for Automotive Mechanical Design Process');
#17359=PRODUCT_CONTEXT('part definition',#17358,'mechanical');
#17366=PRODUCT('Bearing pedestal (1)','Bearing pedestal (1)',
'Bearing pedestal (1)',(#17359));
#17481=COLOUR_RGB('Grey',0.48,0.52,0.57);
#17482=FILL_AREA_STYLE_COLOUR('',#17481);
#17483=FILL_AREA_STYLE('',(#17482));
#17484=SURFACE_STYLE_FILL_AREA(#17483);
#17485=SURFACE_SIDE_STYLE('',(#17484));
#17486=SURFACE_STYLE_USAGE(.BOTH.,#17485);
#17487=PRESENTATION_STYLE_ASSIGNMENT((#17486));
ENDSEC;
END-ISO-10303-21;
